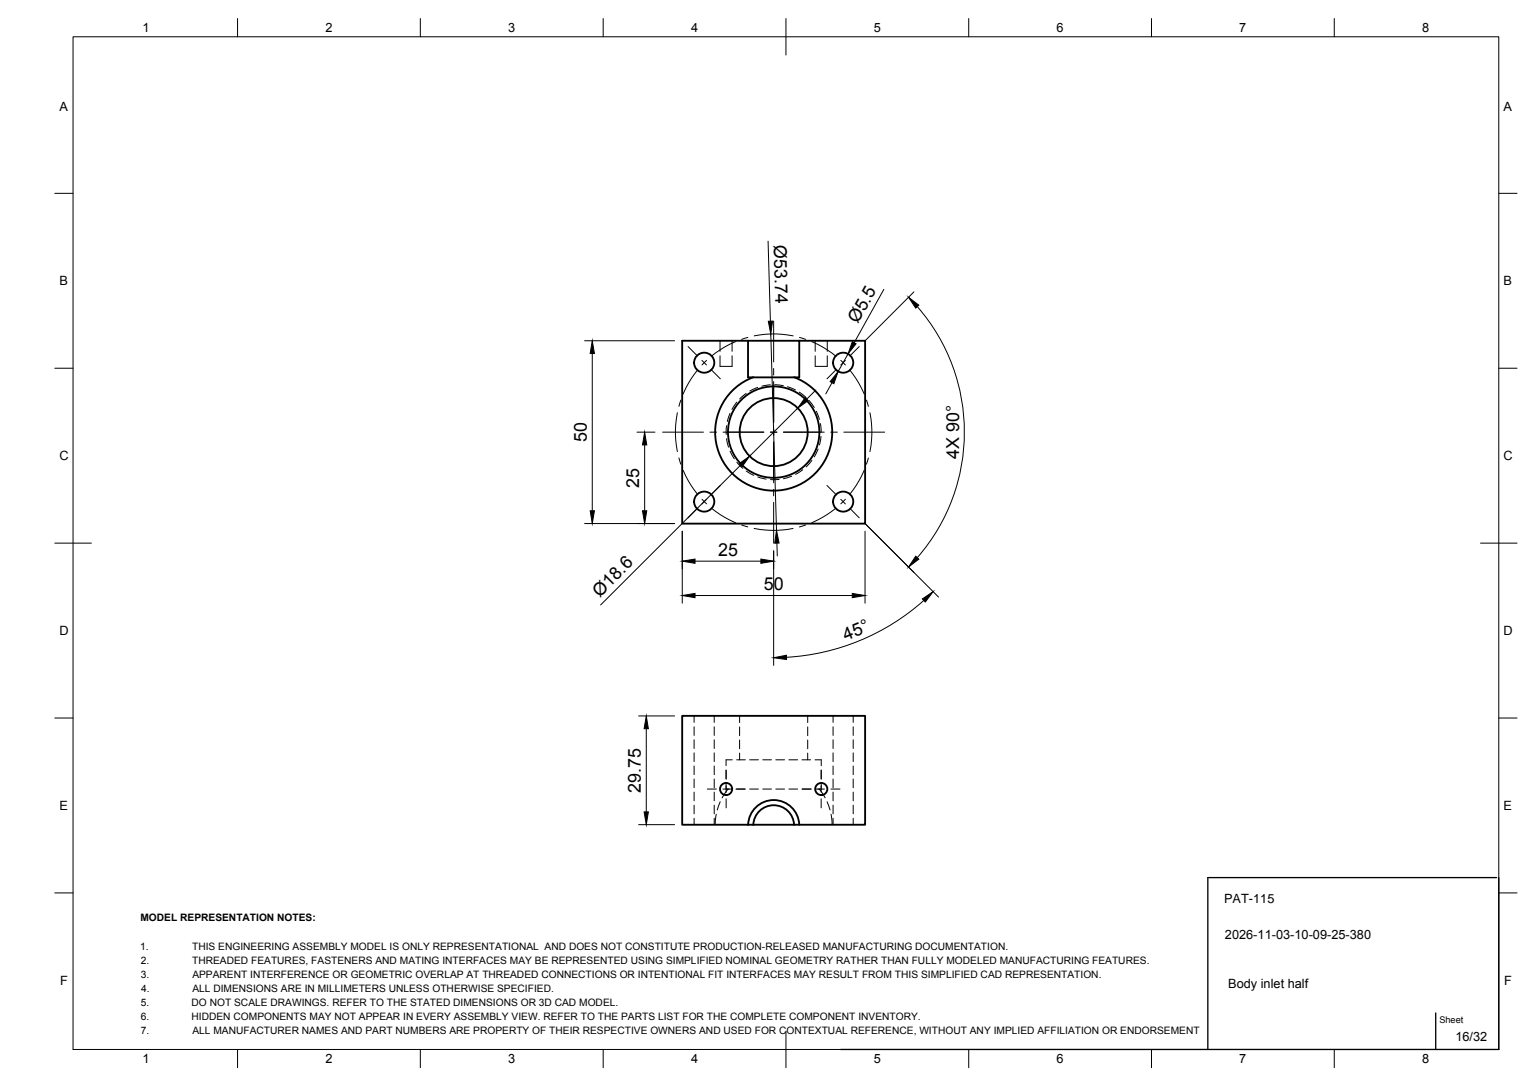
ISO-10303-21;
HEADER;
/* Generated by software containing ST-Developer
 * from STEP Tools, Inc. (www.steptools.com) 
 */

FILE_DESCRIPTION(
/* description */ ('Union bypass pipe loop'),
/* implementation_level */ '2;1');

FILE_NAME(
/* name */ 'Body inlet half.step',
/* time_stamp */ '2026-10-27T21:00:29-07:00',
/* author */ (''),
/* organization */ (''),
/* preprocessor_version */ 'ST-DEVELOPER v20.2',
/* originating_system */ 'Autodesk Translation Framework v15.17.0.0',
/* authorisation */ '');

FILE_SCHEMA (('AUTOMOTIVE_DESIGN { 1 0 10303 214 3 1 1 }'));
ENDSEC;

DATA;
#10=MECHANICAL_DESIGN_GEOMETRIC_PRESENTATION_REPRESENTATION('',(#445),#10095);
#381=SHAPE_REPRESENTATION_RELATIONSHIP('SRR','None',#10250,#413);
#413=ADVANCED_BREP_SHAPE_REPRESENTATION('',(#477),#10062);
#445=STYLED_ITEM('',(#10479),#477);
#477=MANIFOLD_SOLID_BREP('Body1',#5516);
#505=SPHERICAL_SURFACE('',#5944,1.6);
#511=FACE_BOUND('',#1178,.T.);
#512=FACE_BOUND('',#1179,.T.);
#513=FACE_BOUND('',#1183,.T.);
#514=FACE_BOUND('',#1185,.T.);
#515=FACE_BOUND('',#1187,.T.);
#516=FACE_BOUND('',#1189,.T.);
#517=FACE_BOUND('',#1190,.T.);
#518=FACE_BOUND('',#1191,.T.);
#519=FACE_BOUND('',#1192,.T.);
#520=FACE_BOUND('',#1195,.T.);
#521=FACE_BOUND('',#1196,.T.);
#522=FACE_BOUND('',#1197,.T.);
#523=FACE_BOUND('',#1198,.T.);
#524=FACE_BOUND('',#1199,.T.);
#635=PLANE('',#5912);
#636=PLANE('',#5916);
#637=PLANE('',#5932);
#638=PLANE('',#5934);
#639=PLANE('',#5941);
#640=PLANE('',#5943);
#641=PLANE('',#5946);
#642=PLANE('',#5947);
#643=PLANE('',#5948);
#644=PLANE('',#5949);
#645=PLANE('',#5950);
#835=FACE_OUTER_BOUND('',#1167,.T.);
#836=FACE_OUTER_BOUND('',#1168,.T.);
#837=FACE_OUTER_BOUND('',#1169,.T.);
#838=FACE_OUTER_BOUND('',#1170,.T.);
#839=FACE_OUTER_BOUND('',#1171,.T.);
#840=FACE_OUTER_BOUND('',#1172,.T.);
#841=FACE_OUTER_BOUND('',#1173,.T.);
#842=FACE_OUTER_BOUND('',#1174,.T.);
#843=FACE_OUTER_BOUND('',#1175,.T.);
#844=FACE_OUTER_BOUND('',#1176,.T.);
#845=FACE_OUTER_BOUND('',#1177,.T.);
#846=FACE_OUTER_BOUND('',#1180,.T.);
#847=FACE_OUTER_BOUND('',#1181,.T.);
#848=FACE_OUTER_BOUND('',#1182,.T.);
#849=FACE_OUTER_BOUND('',#1184,.T.);
#850=FACE_OUTER_BOUND('',#1186,.T.);
#851=FACE_OUTER_BOUND('',#1188,.T.);
#852=FACE_OUTER_BOUND('',#1193,.T.);
#853=FACE_OUTER_BOUND('',#1194,.T.);
#854=FACE_OUTER_BOUND('',#1200,.T.);
#855=FACE_OUTER_BOUND('',#1201,.T.);
#1167=EDGE_LOOP('',(#3738,#3739,#3740,#3741));
#1168=EDGE_LOOP('',(#3742));
#1169=EDGE_LOOP('',(#3743,#3744,#3745,#3746));
#1170=EDGE_LOOP('',(#3747));
#1171=EDGE_LOOP('',(#3748,#3749,#3750,#3751));
#1172=EDGE_LOOP('',(#3752,#3753,#3754,#3755));
#1173=EDGE_LOOP('',(#3756,#3757,#3758,#3759));
#1174=EDGE_LOOP('',(#3760,#3761,#3762,#3763));
#1175=EDGE_LOOP('',(#3764,#3765,#3766,#3767));
#1176=EDGE_LOOP('',(#3768,#3769,#3770,#3771));
#1177=EDGE_LOOP('',(#3772,#3773,#3774,#3775,#3776,#3777));
#1178=EDGE_LOOP('',(#3778));
#1179=EDGE_LOOP('',(#3779));
#1180=EDGE_LOOP('',(#3780,#3781,#3782,#3783));
#1181=EDGE_LOOP('',(#3784,#3785,#3786,#3787));
#1182=EDGE_LOOP('',(#3788));
#1183=EDGE_LOOP('',(#3789));
#1184=EDGE_LOOP('',(#3790));
#1185=EDGE_LOOP('',(#3791));
#1186=EDGE_LOOP('',(#3792,#3793));
#1187=EDGE_LOOP('',(#3794));
#1188=EDGE_LOOP('',(#3795,#3796,#3797,#3798,#3799,#3800,#3801,#3802,#3803,
#3804));
#1189=EDGE_LOOP('',(#3805));
#1190=EDGE_LOOP('',(#3806));
#1191=EDGE_LOOP('',(#3807));
#1192=EDGE_LOOP('',(#3808));
#1193=EDGE_LOOP('',(#3809,#3810,#3811,#3812));
#1194=EDGE_LOOP('',(#3813,#3814,#3815,#3816));
#1195=EDGE_LOOP('',(#3817));
#1196=EDGE_LOOP('',(#3818));
#1197=EDGE_LOOP('',(#3819));
#1198=EDGE_LOOP('',(#3820));
#1199=EDGE_LOOP('',(#3821));
#1200=EDGE_LOOP('',(#3822,#3823,#3824,#3825));
#1201=EDGE_LOOP('',(#3826,#3827,#3828,#3829));
#1623=LINE('',#8431,#1999);
#1624=LINE('',#8438,#2000);
#1625=LINE('',#8445,#2001);
#1626=LINE('',#8451,#2002);
#1627=LINE('',#8457,#2003);
#1628=LINE('',#8463,#2004);
#1629=LINE('',#8468,#2005);
#1630=LINE('',#8472,#2006);
#1631=LINE('',#8476,#2007);
#1632=LINE('',#8479,#2008);
#1633=LINE('',#8482,#2009);
#1634=LINE('',#8484,#2010);
#1635=LINE('',#8486,#2011);
#1636=LINE('',#8488,#2012);
#1637=LINE('',#8489,#2013);
#1638=LINE('',#8494,#2014);
#1639=LINE('',#8500,#2015);
#1640=LINE('',#8510,#2016);
#1641=LINE('',#8512,#2017);
#1642=LINE('',#8513,#2018);
#1643=LINE('',#8516,#2019);
#1644=LINE('',#8517,#2020);
#1645=LINE('',#8520,#2021);
#1646=LINE('',#8521,#2022);
#1647=LINE('',#8523,#2023);
#1999=VECTOR('',#6631,0.165);
#2000=VECTOR('',#6640,0.165);
#2001=VECTOR('',#6649,0.275);
#2002=VECTOR('',#6656,0.275);
#2003=VECTOR('',#6663,0.275);
#2004=VECTOR('',#6670,0.275);
#2005=VECTOR('',#6675,1.);
#2006=VECTOR('',#6678,1.);
#2007=VECTOR('',#6683,1.);
#2008=VECTOR('',#6686,1.);
#2009=VECTOR('',#6689,1.);
#2010=VECTOR('',#6690,1.);
#2011=VECTOR('',#6691,1.);
#2012=VECTOR('',#6692,1.);
#2013=VECTOR('',#6693,1.);
#2014=VECTOR('',#6698,0.93);
#2015=VECTOR('',#6705,1.3);
#2016=VECTOR('',#6720,1.);
#2017=VECTOR('',#6721,1.);
#2018=VECTOR('',#6722,1.);
#2019=VECTOR('',#6725,1.);
#2020=VECTOR('',#6726,1.);
#2021=VECTOR('',#6729,1.);
#2022=VECTOR('',#6730,1.);
#2023=VECTOR('',#6733,1.);
#2375=CIRCLE('',#5910,0.165);
#2376=CIRCLE('',#5911,0.165);
#2377=CIRCLE('',#5914,0.165);
#2378=CIRCLE('',#5915,0.165);
#2379=CIRCLE('',#5918,0.275);
#2380=CIRCLE('',#5919,0.275);
#2381=CIRCLE('',#5921,0.275);
#2382=CIRCLE('',#5922,0.275);
#2383=CIRCLE('',#5924,0.275);
#2384=CIRCLE('',#5925,0.275);
#2385=CIRCLE('',#5927,0.275);
#2386=CIRCLE('',#5928,0.275);
#2387=CIRCLE('',#5930,0.7);
#2388=CIRCLE('',#5931,0.7);
#2389=CIRCLE('',#5933,0.556776436283003);
#2390=CIRCLE('',#5936,0.93);
#2391=CIRCLE('',#5937,0.93);
#2392=CIRCLE('',#5939,1.3);
#2393=CIRCLE('',#5940,1.3);
#2394=CIRCLE('',#5942,1.24899959967968);
#2395=CIRCLE('',#5945,1.59980467557762);
#2630=VERTEX_POINT('',#8428);
#2631=VERTEX_POINT('',#8430);
#2632=VERTEX_POINT('',#8435);
#2633=VERTEX_POINT('',#8437);
#2634=VERTEX_POINT('',#8442);
#2635=VERTEX_POINT('',#8444);
#2636=VERTEX_POINT('',#8448);
#2637=VERTEX_POINT('',#8450);
#2638=VERTEX_POINT('',#8454);
#2639=VERTEX_POINT('',#8456);
#2640=VERTEX_POINT('',#8460);
#2641=VERTEX_POINT('',#8462);
#2642=VERTEX_POINT('',#8466);
#2643=VERTEX_POINT('',#8467);
#2644=VERTEX_POINT('',#8469);
#2645=VERTEX_POINT('',#8471);
#2646=VERTEX_POINT('',#8475);
#2647=VERTEX_POINT('',#8477);
#2648=VERTEX_POINT('',#8481);
#2649=VERTEX_POINT('',#8483);
#2650=VERTEX_POINT('',#8485);
#2651=VERTEX_POINT('',#8487);
#2652=VERTEX_POINT('',#8491);
#2653=VERTEX_POINT('',#8493);
#2654=VERTEX_POINT('',#8497);
#2655=VERTEX_POINT('',#8499);
#2656=VERTEX_POINT('',#8503);
#2657=VERTEX_POINT('',#8509);
#2658=VERTEX_POINT('',#8511);
#2659=VERTEX_POINT('',#8515);
#2660=VERTEX_POINT('',#8519);
#3067=EDGE_CURVE('',#2630,#2630,#2375,.T.);
#3068=EDGE_CURVE('',#2630,#2631,#1623,.T.);
#3069=EDGE_CURVE('',#2631,#2631,#2376,.T.);
#3070=EDGE_CURVE('',#2632,#2632,#2377,.T.);
#3071=EDGE_CURVE('',#2632,#2633,#1624,.T.);
#3072=EDGE_CURVE('',#2633,#2633,#2378,.T.);
#3073=EDGE_CURVE('',#2634,#2634,#2379,.T.);
#3074=EDGE_CURVE('',#2634,#2635,#1625,.T.);
#3075=EDGE_CURVE('',#2635,#2635,#2380,.T.);
#3076=EDGE_CURVE('',#2636,#2636,#2381,.T.);
#3077=EDGE_CURVE('',#2636,#2637,#1626,.T.);
#3078=EDGE_CURVE('',#2637,#2637,#2382,.T.);
#3079=EDGE_CURVE('',#2638,#2638,#2383,.T.);
#3080=EDGE_CURVE('',#2638,#2639,#1627,.T.);
#3081=EDGE_CURVE('',#2639,#2639,#2384,.T.);
#3082=EDGE_CURVE('',#2640,#2640,#2385,.T.);
#3083=EDGE_CURVE('',#2640,#2641,#1628,.T.);
#3084=EDGE_CURVE('',#2641,#2641,#2386,.T.);
#3085=EDGE_CURVE('',#2642,#2643,#1629,.T.);
#3086=EDGE_CURVE('',#2644,#2642,#2387,.T.);
#3087=EDGE_CURVE('',#2645,#2644,#1630,.T.);
#3088=EDGE_CURVE('',#2643,#2645,#2388,.T.);
#3089=EDGE_CURVE('',#2646,#2642,#1631,.T.);
#3090=EDGE_CURVE('',#2647,#2646,#2389,.T.);
#3091=EDGE_CURVE('',#2644,#2647,#1632,.T.);
#3092=EDGE_CURVE('',#2645,#2648,#1633,.T.);
#3093=EDGE_CURVE('',#2648,#2649,#1634,.T.);
#3094=EDGE_CURVE('',#2649,#2650,#1635,.T.);
#3095=EDGE_CURVE('',#2650,#2651,#1636,.T.);
#3096=EDGE_CURVE('',#2651,#2643,#1637,.T.);
#3097=EDGE_CURVE('',#2652,#2652,#2390,.T.);
#3098=EDGE_CURVE('',#2652,#2653,#1638,.T.);
#3099=EDGE_CURVE('',#2653,#2653,#2391,.T.);
#3100=EDGE_CURVE('',#2654,#2654,#2392,.T.);
#3101=EDGE_CURVE('',#2654,#2655,#1639,.T.);
#3102=EDGE_CURVE('',#2655,#2655,#2393,.T.);
#3103=EDGE_CURVE('',#2656,#2656,#2394,.T.);
#3104=EDGE_CURVE('',#2647,#2646,#2395,.T.);
#3105=EDGE_CURVE('',#2657,#2651,#1640,.T.);
#3106=EDGE_CURVE('',#2657,#2658,#1641,.T.);
#3107=EDGE_CURVE('',#2658,#2648,#1642,.T.);
#3108=EDGE_CURVE('',#2659,#2657,#1643,.T.);
#3109=EDGE_CURVE('',#2659,#2650,#1644,.T.);
#3110=EDGE_CURVE('',#2660,#2659,#1645,.T.);
#3111=EDGE_CURVE('',#2660,#2649,#1646,.T.);
#3112=EDGE_CURVE('',#2658,#2660,#1647,.T.);
#3738=ORIENTED_EDGE('',*,*,#3067,.F.);
#3739=ORIENTED_EDGE('',*,*,#3068,.T.);
#3740=ORIENTED_EDGE('',*,*,#3069,.F.);
#3741=ORIENTED_EDGE('',*,*,#3068,.F.);
#3742=ORIENTED_EDGE('',*,*,#3067,.T.);
#3743=ORIENTED_EDGE('',*,*,#3070,.F.);
#3744=ORIENTED_EDGE('',*,*,#3071,.T.);
#3745=ORIENTED_EDGE('',*,*,#3072,.F.);
#3746=ORIENTED_EDGE('',*,*,#3071,.F.);
#3747=ORIENTED_EDGE('',*,*,#3070,.T.);
#3748=ORIENTED_EDGE('',*,*,#3073,.F.);
#3749=ORIENTED_EDGE('',*,*,#3074,.T.);
#3750=ORIENTED_EDGE('',*,*,#3075,.F.);
#3751=ORIENTED_EDGE('',*,*,#3074,.F.);
#3752=ORIENTED_EDGE('',*,*,#3076,.F.);
#3753=ORIENTED_EDGE('',*,*,#3077,.T.);
#3754=ORIENTED_EDGE('',*,*,#3078,.F.);
#3755=ORIENTED_EDGE('',*,*,#3077,.F.);
#3756=ORIENTED_EDGE('',*,*,#3079,.F.);
#3757=ORIENTED_EDGE('',*,*,#3080,.T.);
#3758=ORIENTED_EDGE('',*,*,#3081,.F.);
#3759=ORIENTED_EDGE('',*,*,#3080,.F.);
#3760=ORIENTED_EDGE('',*,*,#3082,.F.);
#3761=ORIENTED_EDGE('',*,*,#3083,.T.);
#3762=ORIENTED_EDGE('',*,*,#3084,.F.);
#3763=ORIENTED_EDGE('',*,*,#3083,.F.);
#3764=ORIENTED_EDGE('',*,*,#3085,.F.);
#3765=ORIENTED_EDGE('',*,*,#3086,.F.);
#3766=ORIENTED_EDGE('',*,*,#3087,.F.);
#3767=ORIENTED_EDGE('',*,*,#3088,.F.);
#3768=ORIENTED_EDGE('',*,*,#3089,.F.);
#3769=ORIENTED_EDGE('',*,*,#3090,.F.);
#3770=ORIENTED_EDGE('',*,*,#3091,.F.);
#3771=ORIENTED_EDGE('',*,*,#3086,.T.);
#3772=ORIENTED_EDGE('',*,*,#3088,.T.);
#3773=ORIENTED_EDGE('',*,*,#3092,.T.);
#3774=ORIENTED_EDGE('',*,*,#3093,.T.);
#3775=ORIENTED_EDGE('',*,*,#3094,.T.);
#3776=ORIENTED_EDGE('',*,*,#3095,.T.);
#3777=ORIENTED_EDGE('',*,*,#3096,.T.);
#3778=ORIENTED_EDGE('',*,*,#3069,.T.);
#3779=ORIENTED_EDGE('',*,*,#3072,.T.);
#3780=ORIENTED_EDGE('',*,*,#3097,.F.);
#3781=ORIENTED_EDGE('',*,*,#3098,.T.);
#3782=ORIENTED_EDGE('',*,*,#3099,.F.);
#3783=ORIENTED_EDGE('',*,*,#3098,.F.);
#3784=ORIENTED_EDGE('',*,*,#3100,.F.);
#3785=ORIENTED_EDGE('',*,*,#3101,.T.);
#3786=ORIENTED_EDGE('',*,*,#3102,.T.);
#3787=ORIENTED_EDGE('',*,*,#3101,.F.);
#3788=ORIENTED_EDGE('',*,*,#3102,.F.);
#3789=ORIENTED_EDGE('',*,*,#3103,.F.);
#3790=ORIENTED_EDGE('',*,*,#3100,.T.);
#3791=ORIENTED_EDGE('',*,*,#3099,.T.);
#3792=ORIENTED_EDGE('',*,*,#3090,.T.);
#3793=ORIENTED_EDGE('',*,*,#3104,.F.);
#3794=ORIENTED_EDGE('',*,*,#3103,.T.);
#3795=ORIENTED_EDGE('',*,*,#3085,.T.);
#3796=ORIENTED_EDGE('',*,*,#3096,.F.);
#3797=ORIENTED_EDGE('',*,*,#3105,.F.);
#3798=ORIENTED_EDGE('',*,*,#3106,.T.);
#3799=ORIENTED_EDGE('',*,*,#3107,.T.);
#3800=ORIENTED_EDGE('',*,*,#3092,.F.);
#3801=ORIENTED_EDGE('',*,*,#3087,.T.);
#3802=ORIENTED_EDGE('',*,*,#3091,.T.);
#3803=ORIENTED_EDGE('',*,*,#3104,.T.);
#3804=ORIENTED_EDGE('',*,*,#3089,.T.);
#3805=ORIENTED_EDGE('',*,*,#3075,.T.);
#3806=ORIENTED_EDGE('',*,*,#3078,.T.);
#3807=ORIENTED_EDGE('',*,*,#3081,.T.);
#3808=ORIENTED_EDGE('',*,*,#3084,.T.);
#3809=ORIENTED_EDGE('',*,*,#3108,.T.);
#3810=ORIENTED_EDGE('',*,*,#3105,.T.);
#3811=ORIENTED_EDGE('',*,*,#3095,.F.);
#3812=ORIENTED_EDGE('',*,*,#3109,.F.);
#3813=ORIENTED_EDGE('',*,*,#3110,.T.);
#3814=ORIENTED_EDGE('',*,*,#3109,.T.);
#3815=ORIENTED_EDGE('',*,*,#3094,.F.);
#3816=ORIENTED_EDGE('',*,*,#3111,.F.);
#3817=ORIENTED_EDGE('',*,*,#3097,.T.);
#3818=ORIENTED_EDGE('',*,*,#3082,.T.);
#3819=ORIENTED_EDGE('',*,*,#3079,.T.);
#3820=ORIENTED_EDGE('',*,*,#3076,.T.);
#3821=ORIENTED_EDGE('',*,*,#3073,.T.);
#3822=ORIENTED_EDGE('',*,*,#3112,.T.);
#3823=ORIENTED_EDGE('',*,*,#3111,.T.);
#3824=ORIENTED_EDGE('',*,*,#3093,.F.);
#3825=ORIENTED_EDGE('',*,*,#3107,.F.);
#3826=ORIENTED_EDGE('',*,*,#3112,.F.);
#3827=ORIENTED_EDGE('',*,*,#3106,.F.);
#3828=ORIENTED_EDGE('',*,*,#3108,.F.);
#3829=ORIENTED_EDGE('',*,*,#3110,.F.);
#5080=CYLINDRICAL_SURFACE('',#5909,0.165);
#5081=CYLINDRICAL_SURFACE('',#5913,0.165);
#5082=CYLINDRICAL_SURFACE('',#5917,0.275);
#5083=CYLINDRICAL_SURFACE('',#5920,0.275);
#5084=CYLINDRICAL_SURFACE('',#5923,0.275);
#5085=CYLINDRICAL_SURFACE('',#5926,0.275);
#5086=CYLINDRICAL_SURFACE('',#5929,0.7);
#5087=CYLINDRICAL_SURFACE('',#5935,0.93);
#5088=CYLINDRICAL_SURFACE('',#5938,1.3);
#5184=ADVANCED_FACE('',(#835),#5080,.F.);
#5185=ADVANCED_FACE('',(#836),#635,.T.);
#5186=ADVANCED_FACE('',(#837),#5081,.F.);
#5187=ADVANCED_FACE('',(#838),#636,.T.);
#5188=ADVANCED_FACE('',(#839),#5082,.F.);
#5189=ADVANCED_FACE('',(#840),#5083,.F.);
#5190=ADVANCED_FACE('',(#841),#5084,.F.);
#5191=ADVANCED_FACE('',(#842),#5085,.F.);
#5192=ADVANCED_FACE('',(#843),#5086,.F.);
#5193=ADVANCED_FACE('',(#844),#637,.T.);
#5194=ADVANCED_FACE('',(#845,#511,#512),#638,.T.);
#5195=ADVANCED_FACE('',(#846),#5087,.F.);
#5196=ADVANCED_FACE('',(#847),#5088,.F.);
#5197=ADVANCED_FACE('',(#848,#513),#639,.F.);
#5198=ADVANCED_FACE('',(#849,#514),#640,.T.);
#5199=ADVANCED_FACE('',(#850,#515),#505,.F.);
#5200=ADVANCED_FACE('',(#851,#516,#517,#518,#519),#641,.T.);
#5201=ADVANCED_FACE('',(#852),#642,.T.);
#5202=ADVANCED_FACE('',(#853,#520,#521,#522,#523,#524),#643,.T.);
#5203=ADVANCED_FACE('',(#854),#644,.T.);
#5204=ADVANCED_FACE('',(#855),#645,.F.);
#5516=CLOSED_SHELL('',(#5184,#5185,#5186,#5187,#5188,#5189,#5190,#5191,
#5192,#5193,#5194,#5195,#5196,#5197,#5198,#5199,#5200,#5201,#5202,#5203,
#5204));
#5908=AXIS2_PLACEMENT_3D('',#8426,#6625,#6626);
#5909=AXIS2_PLACEMENT_3D('',#8427,#6627,#6628);
#5910=AXIS2_PLACEMENT_3D('',#8429,#6629,#6630);
#5911=AXIS2_PLACEMENT_3D('',#8432,#6632,#6633);
#5912=AXIS2_PLACEMENT_3D('',#8433,#6634,#6635);
#5913=AXIS2_PLACEMENT_3D('',#8434,#6636,#6637);
#5914=AXIS2_PLACEMENT_3D('',#8436,#6638,#6639);
#5915=AXIS2_PLACEMENT_3D('',#8439,#6641,#6642);
#5916=AXIS2_PLACEMENT_3D('',#8440,#6643,#6644);
#5917=AXIS2_PLACEMENT_3D('',#8441,#6645,#6646);
#5918=AXIS2_PLACEMENT_3D('',#8443,#6647,#6648);
#5919=AXIS2_PLACEMENT_3D('',#8446,#6650,#6651);
#5920=AXIS2_PLACEMENT_3D('',#8447,#6652,#6653);
#5921=AXIS2_PLACEMENT_3D('',#8449,#6654,#6655);
#5922=AXIS2_PLACEMENT_3D('',#8452,#6657,#6658);
#5923=AXIS2_PLACEMENT_3D('',#8453,#6659,#6660);
#5924=AXIS2_PLACEMENT_3D('',#8455,#6661,#6662);
#5925=AXIS2_PLACEMENT_3D('',#8458,#6664,#6665);
#5926=AXIS2_PLACEMENT_3D('',#8459,#6666,#6667);
#5927=AXIS2_PLACEMENT_3D('',#8461,#6668,#6669);
#5928=AXIS2_PLACEMENT_3D('',#8464,#6671,#6672);
#5929=AXIS2_PLACEMENT_3D('',#8465,#6673,#6674);
#5930=AXIS2_PLACEMENT_3D('',#8470,#6676,#6677);
#5931=AXIS2_PLACEMENT_3D('',#8473,#6679,#6680);
#5932=AXIS2_PLACEMENT_3D('',#8474,#6681,#6682);
#5933=AXIS2_PLACEMENT_3D('',#8478,#6684,#6685);
#5934=AXIS2_PLACEMENT_3D('',#8480,#6687,#6688);
#5935=AXIS2_PLACEMENT_3D('',#8490,#6694,#6695);
#5936=AXIS2_PLACEMENT_3D('',#8492,#6696,#6697);
#5937=AXIS2_PLACEMENT_3D('',#8495,#6699,#6700);
#5938=AXIS2_PLACEMENT_3D('',#8496,#6701,#6702);
#5939=AXIS2_PLACEMENT_3D('',#8498,#6703,#6704);
#5940=AXIS2_PLACEMENT_3D('',#8501,#6706,#6707);
#5941=AXIS2_PLACEMENT_3D('',#8502,#6708,#6709);
#5942=AXIS2_PLACEMENT_3D('',#8504,#6710,#6711);
#5943=AXIS2_PLACEMENT_3D('',#8505,#6712,#6713);
#5944=AXIS2_PLACEMENT_3D('',#8506,#6714,#6715);
#5945=AXIS2_PLACEMENT_3D('',#8507,#6716,#6717);
#5946=AXIS2_PLACEMENT_3D('',#8508,#6718,#6719);
#5947=AXIS2_PLACEMENT_3D('',#8514,#6723,#6724);
#5948=AXIS2_PLACEMENT_3D('',#8518,#6727,#6728);
#5949=AXIS2_PLACEMENT_3D('',#8522,#6731,#6732);
#5950=AXIS2_PLACEMENT_3D('',#8524,#6734,#6735);
#6625=DIRECTION('axis',(0.,0.,1.));
#6626=DIRECTION('refdir',(1.,0.,0.));
#6627=DIRECTION('center_axis',(0.,0.,1.));
#6628=DIRECTION('ref_axis',(1.,0.,0.));
#6629=DIRECTION('center_axis',(0.,0.,1.));
#6630=DIRECTION('ref_axis',(1.,0.,0.));
#6631=DIRECTION('',(0.,0.,1.));
#6632=DIRECTION('center_axis',(0.,0.,-1.));
#6633=DIRECTION('ref_axis',(1.,0.,0.));
#6634=DIRECTION('center_axis',(0.,0.,1.));
#6635=DIRECTION('ref_axis',(1.,0.,0.));
#6636=DIRECTION('center_axis',(0.,0.,1.));
#6637=DIRECTION('ref_axis',(1.,0.,0.));
#6638=DIRECTION('center_axis',(0.,0.,1.));
#6639=DIRECTION('ref_axis',(1.,0.,0.));
#6640=DIRECTION('',(0.,0.,1.));
#6641=DIRECTION('center_axis',(0.,0.,-1.));
#6642=DIRECTION('ref_axis',(1.,0.,0.));
#6643=DIRECTION('center_axis',(0.,0.,1.));
#6644=DIRECTION('ref_axis',(1.,0.,0.));
#6645=DIRECTION('center_axis',(0.,1.,0.));
#6646=DIRECTION('ref_axis',(1.,0.,0.));
#6647=DIRECTION('center_axis',(0.,1.,0.));
#6648=DIRECTION('ref_axis',(1.,0.,0.));
#6649=DIRECTION('',(0.,1.,0.));
#6650=DIRECTION('center_axis',(0.,-1.,0.));
#6651=DIRECTION('ref_axis',(1.,0.,0.));
#6652=DIRECTION('center_axis',(0.,1.,0.));
#6653=DIRECTION('ref_axis',(1.,0.,0.));
#6654=DIRECTION('center_axis',(0.,1.,0.));
#6655=DIRECTION('ref_axis',(1.,0.,0.));
#6656=DIRECTION('',(0.,1.,0.));
#6657=DIRECTION('center_axis',(0.,-1.,0.));
#6658=DIRECTION('ref_axis',(1.,0.,0.));
#6659=DIRECTION('center_axis',(0.,1.,0.));
#6660=DIRECTION('ref_axis',(1.,0.,0.));
#6661=DIRECTION('center_axis',(0.,1.,0.));
#6662=DIRECTION('ref_axis',(1.,0.,0.));
#6663=DIRECTION('',(0.,1.,0.));
#6664=DIRECTION('center_axis',(0.,-1.,0.));
#6665=DIRECTION('ref_axis',(1.,0.,0.));
#6666=DIRECTION('center_axis',(0.,1.,0.));
#6667=DIRECTION('ref_axis',(1.,0.,0.));
#6668=DIRECTION('center_axis',(0.,1.,0.));
#6669=DIRECTION('ref_axis',(1.,0.,0.));
#6670=DIRECTION('',(0.,1.,0.));
#6671=DIRECTION('center_axis',(0.,-1.,0.));
#6672=DIRECTION('ref_axis',(1.,0.,0.));
#6673=DIRECTION('center_axis',(0.,0.,1.));
#6674=DIRECTION('ref_axis',(1.,0.,0.));
#6675=DIRECTION('',(0.,0.,1.));
#6676=DIRECTION('center_axis',(0.,0.,1.));
#6677=DIRECTION('ref_axis',(1.,0.,0.));
#6678=DIRECTION('',(0.,0.,-1.));
#6679=DIRECTION('center_axis',(0.,0.,-1.));
#6680=DIRECTION('ref_axis',(1.,0.,0.));
#6681=DIRECTION('center_axis',(0.,0.,1.));
#6682=DIRECTION('ref_axis',(1.,0.,0.));
#6683=DIRECTION('',(1.,0.,0.));
#6684=DIRECTION('center_axis',(0.,0.,1.));
#6685=DIRECTION('ref_axis',(0.,-1.,0.));
#6686=DIRECTION('',(1.,0.,0.));
#6687=DIRECTION('center_axis',(0.,0.,1.));
#6688=DIRECTION('ref_axis',(1.,0.,0.));
#6689=DIRECTION('',(-1.,0.,0.));
#6690=DIRECTION('',(0.,-1.,0.));
#6691=DIRECTION('',(1.,0.,0.));
#6692=DIRECTION('',(0.,1.,0.));
#6693=DIRECTION('',(-1.,0.,0.));
#6694=DIRECTION('center_axis',(0.,1.,0.));
#6695=DIRECTION('ref_axis',(1.,0.,0.));
#6696=DIRECTION('center_axis',(0.,1.,0.));
#6697=DIRECTION('ref_axis',(1.,0.,0.));
#6698=DIRECTION('',(0.,1.,0.));
#6699=DIRECTION('center_axis',(0.,-1.,0.));
#6700=DIRECTION('ref_axis',(1.,0.,0.));
#6701=DIRECTION('center_axis',(0.,1.,0.));
#6702=DIRECTION('ref_axis',(1.,0.,0.));
#6703=DIRECTION('center_axis',(0.,1.,0.));
#6704=DIRECTION('ref_axis',(1.,0.,0.));
#6705=DIRECTION('',(0.,1.,0.));
#6706=DIRECTION('center_axis',(0.,1.,0.));
#6707=DIRECTION('ref_axis',(1.,0.,0.));
#6708=DIRECTION('center_axis',(0.,1.,0.));
#6709=DIRECTION('ref_axis',(1.,0.,0.));
#6710=DIRECTION('center_axis',(0.,-1.,0.));
#6711=DIRECTION('ref_axis',(0.,0.,-1.));
#6712=DIRECTION('center_axis',(0.,1.,0.));
#6713=DIRECTION('ref_axis',(1.,0.,0.));
#6714=DIRECTION('center_axis',(6.12323399573677E-17,0.,1.));
#6715=DIRECTION('ref_axis',(1.,0.,0.));
#6716=DIRECTION('center_axis',(0.,-1.,0.));
#6717=DIRECTION('ref_axis',(0.,0.,-1.));
#6718=DIRECTION('center_axis',(0.,1.,0.));
#6719=DIRECTION('ref_axis',(-1.,0.,0.));
#6720=DIRECTION('',(0.,0.,1.));
#6721=DIRECTION('',(-1.,0.,0.));
#6722=DIRECTION('',(0.,0.,1.));
#6723=DIRECTION('center_axis',(1.,0.,0.));
#6724=DIRECTION('ref_axis',(0.,1.,0.));
#6725=DIRECTION('',(0.,1.,0.));
#6726=DIRECTION('',(0.,0.,1.));
#6727=DIRECTION('center_axis',(0.,-1.,0.));
#6728=DIRECTION('ref_axis',(1.,0.,0.));
#6729=DIRECTION('',(1.,0.,0.));
#6730=DIRECTION('',(0.,0.,1.));
#6731=DIRECTION('center_axis',(-1.,0.,0.));
#6732=DIRECTION('ref_axis',(0.,-1.,0.));
#6733=DIRECTION('',(0.,-1.,0.));
#6734=DIRECTION('center_axis',(0.,0.,1.));
#6735=DIRECTION('ref_axis',(1.,0.,0.));
#8426=CARTESIAN_POINT('',(0.,0.,0.));
#8427=CARTESIAN_POINT('Origin',(-1.3,-1.,6.8));
#8428=CARTESIAN_POINT('',(-1.465,-1.,6.8));
#8429=CARTESIAN_POINT('Origin',(-1.3,-1.,6.8));
#8430=CARTESIAN_POINT('',(-1.465,-1.,7.5));
#8431=CARTESIAN_POINT('',(-1.465,-1.,6.8));
#8432=CARTESIAN_POINT('Origin',(-1.3,-1.,7.5));
#8433=CARTESIAN_POINT('Origin',(-1.3,-1.,6.8));
#8434=CARTESIAN_POINT('Origin',(1.3,-1.,6.8));
#8435=CARTESIAN_POINT('',(1.135,-1.,6.8));
#8436=CARTESIAN_POINT('Origin',(1.3,-1.,6.8));
#8437=CARTESIAN_POINT('',(1.135,-1.,7.5));
#8438=CARTESIAN_POINT('',(1.135,-1.,6.8));
#8439=CARTESIAN_POINT('Origin',(1.3,-1.,7.5));
#8440=CARTESIAN_POINT('Origin',(1.3,-1.,6.8));
#8441=CARTESIAN_POINT('Origin',(1.9,-3.1,3.1));
#8442=CARTESIAN_POINT('',(1.625,-3.,3.1));
#8443=CARTESIAN_POINT('Origin',(1.9,-3.,3.1));
#8444=CARTESIAN_POINT('',(1.625,-0.0249999999999999,3.1));
#8445=CARTESIAN_POINT('',(1.625,-3.1,3.1));
#8446=CARTESIAN_POINT('Origin',(1.9,-0.0249999999999999,3.1));
#8447=CARTESIAN_POINT('Origin',(-1.9,-3.1,6.9));
#8448=CARTESIAN_POINT('',(-2.175,-3.,6.9));
#8449=CARTESIAN_POINT('Origin',(-1.9,-3.,6.9));
#8450=CARTESIAN_POINT('',(-2.175,-0.0249999999999999,6.9));
#8451=CARTESIAN_POINT('',(-2.175,-3.1,6.9));
#8452=CARTESIAN_POINT('Origin',(-1.9,-0.0249999999999999,6.9));
#8453=CARTESIAN_POINT('Origin',(-1.9,-3.1,3.1));
#8454=CARTESIAN_POINT('',(-2.175,-3.,3.1));
#8455=CARTESIAN_POINT('Origin',(-1.9,-3.,3.1));
#8456=CARTESIAN_POINT('',(-2.175,-0.0249999999999999,3.1));
#8457=CARTESIAN_POINT('',(-2.175,-3.1,3.1));
#8458=CARTESIAN_POINT('Origin',(-1.9,-0.0249999999999999,3.1));
#8459=CARTESIAN_POINT('Origin',(1.9,-3.1,6.9));
#8460=CARTESIAN_POINT('',(1.625,-3.,6.9));
#8461=CARTESIAN_POINT('Origin',(1.9,-3.,6.9));
#8462=CARTESIAN_POINT('',(1.625,-0.0249999999999999,6.9));
#8463=CARTESIAN_POINT('',(1.625,-3.1,6.9));
#8464=CARTESIAN_POINT('Origin',(1.9,-0.0249999999999999,6.9));
#8465=CARTESIAN_POINT('Origin',(0.,0.,6.5));
#8466=CARTESIAN_POINT('',(0.699553428981661,-0.025,6.5));
#8467=CARTESIAN_POINT('',(0.699553428981661,-0.025,7.5));
#8468=CARTESIAN_POINT('',(0.699553428981661,-0.025,6.5));
#8469=CARTESIAN_POINT('',(-0.699553428981661,-0.025,6.5));
#8470=CARTESIAN_POINT('Origin',(0.,0.,6.5));
#8471=CARTESIAN_POINT('',(-0.699553428981661,-0.025,7.5));
#8472=CARTESIAN_POINT('',(-0.699553428981661,-0.025,6.5));
#8473=CARTESIAN_POINT('Origin',(0.,0.,7.5));
#8474=CARTESIAN_POINT('Origin',(0.,0.,6.5));
#8475=CARTESIAN_POINT('',(0.556214886532175,-0.025,6.5));
#8476=CARTESIAN_POINT('',(1.25,-0.025,6.5));
#8477=CARTESIAN_POINT('',(-0.556214886532175,-0.025,6.5));
#8478=CARTESIAN_POINT('Origin',(0.,0.,6.5));
#8479=CARTESIAN_POINT('',(1.25,-0.025,6.5));
#8480=CARTESIAN_POINT('Origin',(0.,-1.5125,7.5));
#8481=CARTESIAN_POINT('',(-2.5,-0.025,7.5));
#8482=CARTESIAN_POINT('',(2.5,-0.025,7.5));
#8483=CARTESIAN_POINT('',(-2.5,-3.,7.5));
#8484=CARTESIAN_POINT('',(-2.5,-0.025,7.5));
#8485=CARTESIAN_POINT('',(2.5,-3.,7.5));
#8486=CARTESIAN_POINT('',(-2.5,-3.,7.5));
#8487=CARTESIAN_POINT('',(2.5,-0.025,7.5));
#8488=CARTESIAN_POINT('',(2.5,-3.,7.5));
#8489=CARTESIAN_POINT('',(2.5,-0.025,7.5));
#8490=CARTESIAN_POINT('Origin',(0.,-3.1,5.));
#8491=CARTESIAN_POINT('',(-0.93,-3.,5.));
#8492=CARTESIAN_POINT('Origin',(0.,-3.,5.));
#8493=CARTESIAN_POINT('',(-0.93,-1.8,5.));
#8494=CARTESIAN_POINT('',(-0.93,-3.1,5.));
#8495=CARTESIAN_POINT('Origin',(0.,-1.8,5.));
#8496=CARTESIAN_POINT('Origin',(0.,-1.8,5.));
#8497=CARTESIAN_POINT('',(-1.3,-1.8,5.));
#8498=CARTESIAN_POINT('Origin',(0.,-1.8,5.));
#8499=CARTESIAN_POINT('',(-1.3,-1.,5.));
#8500=CARTESIAN_POINT('',(-1.3,-1.8,5.));
#8501=CARTESIAN_POINT('Origin',(0.,-1.,5.));
#8502=CARTESIAN_POINT('Origin',(0.,-1.,5.));
#8503=CARTESIAN_POINT('',(-1.52958336188405E-16,-1.,6.24899959967968));
#8504=CARTESIAN_POINT('Origin',(0.,-1.,5.));
#8505=CARTESIAN_POINT('Origin',(0.,-1.8,5.));
#8506=CARTESIAN_POINT('Origin',(0.,0.,5.));
#8507=CARTESIAN_POINT('Origin',(0.,-0.025,5.));
#8508=CARTESIAN_POINT('Origin',(2.5,-0.025,2.5));
#8509=CARTESIAN_POINT('',(2.5,-0.025,2.5));
#8510=CARTESIAN_POINT('',(2.5,-0.025,2.5));
#8511=CARTESIAN_POINT('',(-2.5,-0.025,2.5));
#8512=CARTESIAN_POINT('',(2.5,-0.025,2.5));
#8513=CARTESIAN_POINT('',(-2.5,-0.025,2.5));
#8514=CARTESIAN_POINT('Origin',(2.5,-3.,2.5));
#8515=CARTESIAN_POINT('',(2.5,-3.,2.5));
#8516=CARTESIAN_POINT('',(2.5,-3.,2.5));
#8517=CARTESIAN_POINT('',(2.5,-3.,2.5));
#8518=CARTESIAN_POINT('Origin',(-2.5,-3.,2.5));
#8519=CARTESIAN_POINT('',(-2.5,-3.,2.5));
#8520=CARTESIAN_POINT('',(-2.5,-3.,2.5));
#8521=CARTESIAN_POINT('',(-2.5,-3.,2.5));
#8522=CARTESIAN_POINT('Origin',(-2.5,-0.025,2.5));
#8523=CARTESIAN_POINT('',(-2.5,-0.025,2.5));
#8524=CARTESIAN_POINT('Origin',(0.,-1.5125,2.5));
#10025=UNCERTAINTY_MEASURE_WITH_UNIT(LENGTH_MEASURE(0.001),#10096,
'DISTANCE_ACCURACY_VALUE',
'Maximum model space distance between geometric entities at asserted c
onnectivities');
#10058=UNCERTAINTY_MEASURE_WITH_UNIT(LENGTH_MEASURE(0.001),#10096,
'DISTANCE_ACCURACY_VALUE',
'Maximum model space distance between geometric entities at asserted c
onnectivities');
#10062=(
GEOMETRIC_REPRESENTATION_CONTEXT(3)
GLOBAL_UNCERTAINTY_ASSIGNED_CONTEXT((#10025))
GLOBAL_UNIT_ASSIGNED_CONTEXT((#10096,#10098,#10099))
REPRESENTATION_CONTEXT('','3D')
);
#10095=(
GEOMETRIC_REPRESENTATION_CONTEXT(3)
GLOBAL_UNCERTAINTY_ASSIGNED_CONTEXT((#10058))
GLOBAL_UNIT_ASSIGNED_CONTEXT((#10096,#10098,#10099))
REPRESENTATION_CONTEXT('','3D')
);
#10096=(
LENGTH_UNIT()
NAMED_UNIT(*)
SI_UNIT(.CENTI.,.METRE.)
);
#10098=(
NAMED_UNIT(*)
PLANE_ANGLE_UNIT()
SI_UNIT($,.RADIAN.)
);
#10099=(
NAMED_UNIT(*)
SI_UNIT($,.STERADIAN.)
SOLID_ANGLE_UNIT()
);
#10103=SHAPE_DEFINITION_REPRESENTATION(#10139,#10250);
#10139=PRODUCT_DEFINITION_SHAPE('',$,#10287);
#10250=SHAPE_REPRESENTATION('',(#5908),#10062);
#10283=PRODUCT_DEFINITION_CONTEXT('part definition',#10393,'design');
#10287=PRODUCT_DEFINITION('Body inlet half','Body inlet half',#10323,#10283);
#10323=PRODUCT_DEFINITION_FORMATION('',$,#10398);
#10393=APPLICATION_CONTEXT(
'Core Data for Automotive Mechanical Design Process');
#10394=PRODUCT_CONTEXT('part definition',#10393,'mechanical');
#10398=PRODUCT('Body inlet half','Body inlet half','Body inlet half',(#10394));
#10473=COLOUR_RGB('Dark Blue',0.08,0.2,0.34);
#10474=FILL_AREA_STYLE_COLOUR('',#10473);
#10475=FILL_AREA_STYLE('',(#10474));
#10476=SURFACE_STYLE_FILL_AREA(#10475);
#10477=SURFACE_SIDE_STYLE('',(#10476));
#10478=SURFACE_STYLE_USAGE(.BOTH.,#10477);
#10479=PRESENTATION_STYLE_ASSIGNMENT((#10478));
ENDSEC;
END-ISO-10303-21;
